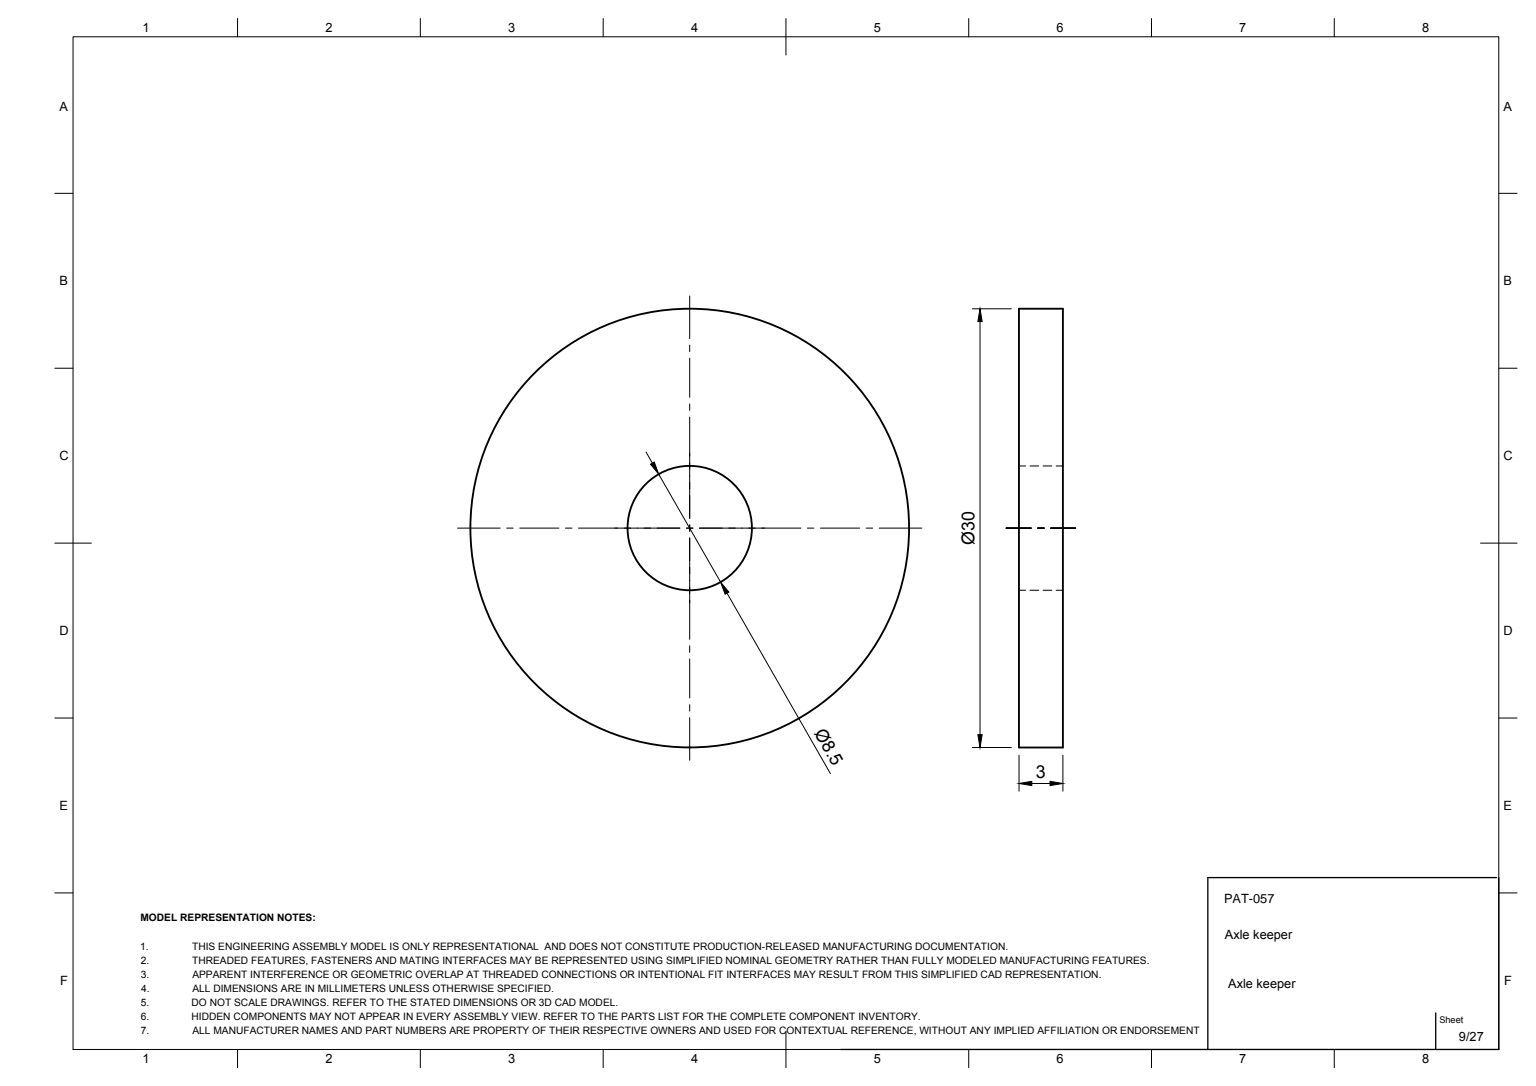
ISO-10303-21;
HEADER;
/* Generated by software containing ST-Developer
 * from STEP Tools, Inc. (www.steptools.com) 
 */

FILE_DESCRIPTION(
/* description */ ('Bearing-mounted hook block'),
/* implementation_level */ '2;1');

FILE_NAME(
/* name */ 'Axle keeper.step',
/* time_stamp */ '2026-10-28T22:30:11-07:00',
/* author */ (''),
/* organization */ (''),
/* preprocessor_version */ 'ST-DEVELOPER v20.2',
/* originating_system */ 'Autodesk Translation Framework v15.17.0.0',
/* authorisation */ '');

FILE_SCHEMA (('AUTOMOTIVE_DESIGN { 1 0 10303 214 3 1 1 }'));
ENDSEC;

DATA;
#10=MECHANICAL_DESIGN_GEOMETRIC_PRESENTATION_REPRESENTATION('',(#327),#7609);
#279=SHAPE_REPRESENTATION_RELATIONSHIP('SRR','None',#7726,#303);
#303=ADVANCED_BREP_SHAPE_REPRESENTATION('',(#359),#7586);
#327=STYLED_ITEM('',(#7931),#359);
#359=MANIFOLD_SOLID_BREP('Body1',#3923);
#445=LINE('',#6304,#675);
#446=LINE('',#6310,#676);
#675=VECTOR('',#5026,0.425);
#676=VECTOR('',#5033,1.5);
#865=CYLINDRICAL_SURFACE('',#4321,0.425);
#866=CYLINDRICAL_SURFACE('',#4324,1.5);
#945=FACE_BOUND('',#1309,.T.);
#946=FACE_BOUND('',#1311,.T.);
#1046=FACE_OUTER_BOUND('',#1306,.T.);
#1047=FACE_OUTER_BOUND('',#1307,.T.);
#1048=FACE_OUTER_BOUND('',#1308,.T.);
#1049=FACE_OUTER_BOUND('',#1310,.T.);
#1306=EDGE_LOOP('',(#2812,#2813,#2814,#2815));
#1307=EDGE_LOOP('',(#2816,#2817,#2818,#2819));
#1308=EDGE_LOOP('',(#2820));
#1309=EDGE_LOOP('',(#2821));
#1310=EDGE_LOOP('',(#2822));
#1311=EDGE_LOOP('',(#2823));
#1603=CIRCLE('',#4322,0.425);
#1604=CIRCLE('',#4323,0.425);
#1605=CIRCLE('',#4325,1.5);
#1606=CIRCLE('',#4326,1.5);
#1852=VERTEX_POINT('',#6301);
#1853=VERTEX_POINT('',#6303);
#1854=VERTEX_POINT('',#6307);
#1855=VERTEX_POINT('',#6309);
#2216=EDGE_CURVE('',#1852,#1852,#1603,.T.);
#2217=EDGE_CURVE('',#1852,#1853,#445,.T.);
#2218=EDGE_CURVE('',#1853,#1853,#1604,.T.);
#2219=EDGE_CURVE('',#1854,#1854,#1605,.T.);
#2220=EDGE_CURVE('',#1854,#1855,#446,.T.);
#2221=EDGE_CURVE('',#1855,#1855,#1606,.T.);
#2812=ORIENTED_EDGE('',*,*,#2216,.F.);
#2813=ORIENTED_EDGE('',*,*,#2217,.T.);
#2814=ORIENTED_EDGE('',*,*,#2218,.T.);
#2815=ORIENTED_EDGE('',*,*,#2217,.F.);
#2816=ORIENTED_EDGE('',*,*,#2219,.F.);
#2817=ORIENTED_EDGE('',*,*,#2220,.T.);
#2818=ORIENTED_EDGE('',*,*,#2221,.T.);
#2819=ORIENTED_EDGE('',*,*,#2220,.F.);
#2820=ORIENTED_EDGE('',*,*,#2219,.T.);
#2821=ORIENTED_EDGE('',*,*,#2216,.T.);
#2822=ORIENTED_EDGE('',*,*,#2221,.F.);
#2823=ORIENTED_EDGE('',*,*,#2218,.F.);
#3584=PLANE('',#4327);
#3585=PLANE('',#4328);
#3728=ADVANCED_FACE('',(#1046),#865,.F.);
#3729=ADVANCED_FACE('',(#1047),#866,.T.);
#3730=ADVANCED_FACE('',(#1048,#945),#3584,.T.);
#3731=ADVANCED_FACE('',(#1049,#946),#3585,.F.);
#3923=CLOSED_SHELL('',(#3728,#3729,#3730,#3731));
#4320=AXIS2_PLACEMENT_3D('',#6299,#5020,#5021);
#4321=AXIS2_PLACEMENT_3D('',#6300,#5022,#5023);
#4322=AXIS2_PLACEMENT_3D('',#6302,#5024,#5025);
#4323=AXIS2_PLACEMENT_3D('',#6305,#5027,#5028);
#4324=AXIS2_PLACEMENT_3D('',#6306,#5029,#5030);
#4325=AXIS2_PLACEMENT_3D('',#6308,#5031,#5032);
#4326=AXIS2_PLACEMENT_3D('',#6311,#5034,#5035);
#4327=AXIS2_PLACEMENT_3D('',#6312,#5036,#5037);
#4328=AXIS2_PLACEMENT_3D('',#6313,#5038,#5039);
#5020=DIRECTION('axis',(0.,0.,1.));
#5021=DIRECTION('refdir',(1.,0.,0.));
#5022=DIRECTION('center_axis',(0.,1.,0.));
#5023=DIRECTION('ref_axis',(1.,0.,0.));
#5024=DIRECTION('center_axis',(0.,-1.,0.));
#5025=DIRECTION('ref_axis',(1.,0.,0.));
#5026=DIRECTION('',(0.,-1.,0.));
#5027=DIRECTION('center_axis',(0.,-1.,0.));
#5028=DIRECTION('ref_axis',(1.,0.,0.));
#5029=DIRECTION('center_axis',(0.,1.,0.));
#5030=DIRECTION('ref_axis',(1.,0.,0.));
#5031=DIRECTION('center_axis',(0.,1.,0.));
#5032=DIRECTION('ref_axis',(1.,0.,0.));
#5033=DIRECTION('',(0.,-1.,0.));
#5034=DIRECTION('center_axis',(0.,1.,0.));
#5035=DIRECTION('ref_axis',(1.,0.,0.));
#5036=DIRECTION('center_axis',(0.,1.,0.));
#5037=DIRECTION('ref_axis',(1.,0.,0.));
#5038=DIRECTION('center_axis',(0.,1.,0.));
#5039=DIRECTION('ref_axis',(1.,0.,0.));
#6299=CARTESIAN_POINT('',(0.,0.,0.));
#6300=CARTESIAN_POINT('Origin',(0.,3.1,12.));
#6301=CARTESIAN_POINT('',(-0.425,3.4,12.));
#6302=CARTESIAN_POINT('Origin',(0.,3.4,12.));
#6303=CARTESIAN_POINT('',(-0.425,3.1,12.));
#6304=CARTESIAN_POINT('',(-0.425,3.1,12.));
#6305=CARTESIAN_POINT('Origin',(0.,3.1,12.));
#6306=CARTESIAN_POINT('Origin',(0.,3.1,12.));
#6307=CARTESIAN_POINT('',(-1.5,3.4,12.));
#6308=CARTESIAN_POINT('Origin',(0.,3.4,12.));
#6309=CARTESIAN_POINT('',(-1.5,3.1,12.));
#6310=CARTESIAN_POINT('',(-1.5,3.1,12.));
#6311=CARTESIAN_POINT('Origin',(0.,3.1,12.));
#6312=CARTESIAN_POINT('Origin',(0.,3.4,12.));
#6313=CARTESIAN_POINT('Origin',(0.,3.1,12.));
#7556=UNCERTAINTY_MEASURE_WITH_UNIT(LENGTH_MEASURE(0.001),#7610,
'DISTANCE_ACCURACY_VALUE',
'Maximum model space distance between geometric entities at asserted c
onnectivities');
#7579=UNCERTAINTY_MEASURE_WITH_UNIT(LENGTH_MEASURE(0.001),#7610,
'DISTANCE_ACCURACY_VALUE',
'Maximum model space distance between geometric entities at asserted c
onnectivities');
#7586=(
GEOMETRIC_REPRESENTATION_CONTEXT(3)
GLOBAL_UNCERTAINTY_ASSIGNED_CONTEXT((#7556))
GLOBAL_UNIT_ASSIGNED_CONTEXT((#7610,#7612,#7613))
REPRESENTATION_CONTEXT('','3D')
);
#7609=(
GEOMETRIC_REPRESENTATION_CONTEXT(3)
GLOBAL_UNCERTAINTY_ASSIGNED_CONTEXT((#7579))
GLOBAL_UNIT_ASSIGNED_CONTEXT((#7610,#7612,#7613))
REPRESENTATION_CONTEXT('','3D')
);
#7610=(
LENGTH_UNIT()
NAMED_UNIT(*)
SI_UNIT(.CENTI.,.METRE.)
);
#7612=(
NAMED_UNIT(*)
PLANE_ANGLE_UNIT()
SI_UNIT($,.RADIAN.)
);
#7613=(
NAMED_UNIT(*)
SI_UNIT($,.STERADIAN.)
SOLID_ANGLE_UNIT()
);
#7620=SHAPE_DEFINITION_REPRESENTATION(#7649,#7726);
#7649=PRODUCT_DEFINITION_SHAPE('',$,#7756);
#7726=SHAPE_REPRESENTATION('',(#4320),#7586);
#7749=PRODUCT_DEFINITION_CONTEXT('part definition',#7838,'design');
#7756=PRODUCT_DEFINITION('Axle keeper','Axle keeper',#7785,#7749);
#7785=PRODUCT_DEFINITION_FORMATION('',$,#7846);
#7838=APPLICATION_CONTEXT(
'Core Data for Automotive Mechanical Design Process');
#7839=PRODUCT_CONTEXT('part definition',#7838,'mechanical');
#7846=PRODUCT('Axle keeper','Axle keeper','Axle keeper',(#7839));
#7925=COLOUR_RGB('Grey',0.48,0.52,0.57);
#7926=FILL_AREA_STYLE_COLOUR('',#7925);
#7927=FILL_AREA_STYLE('',(#7926));
#7928=SURFACE_STYLE_FILL_AREA(#7927);
#7929=SURFACE_SIDE_STYLE('',(#7928));
#7930=SURFACE_STYLE_USAGE(.BOTH.,#7929);
#7931=PRESENTATION_STYLE_ASSIGNMENT((#7930));
ENDSEC;
END-ISO-10303-21;
